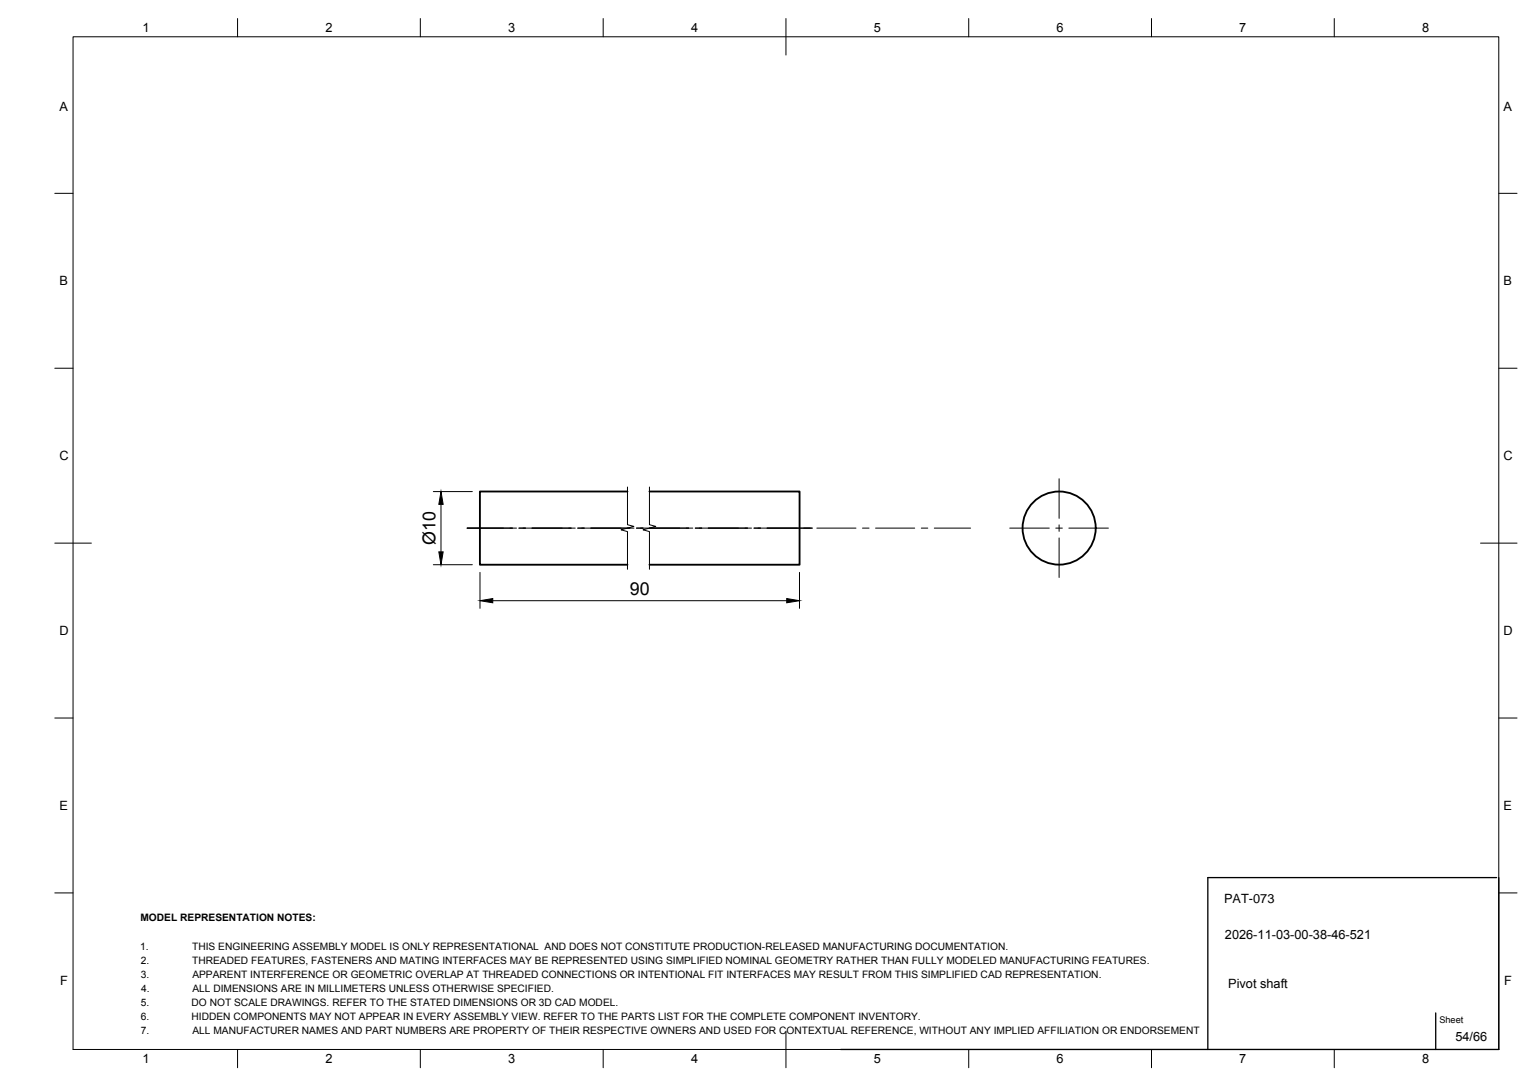
ISO-10303-21;
HEADER;
/* Generated by software containing ST-Developer
 * from STEP Tools, Inc. (www.steptools.com) 
 */

FILE_DESCRIPTION(
/* description */ ('Manual piston pump'),
/* implementation_level */ '2;1');

FILE_NAME(
/* name */ 'Pivot shaft.step',
/* time_stamp */ '2026-11-02T16:54:23-08:00',
/* author */ (''),
/* organization */ (''),
/* preprocessor_version */ 'ST-DEVELOPER v20.2',
/* originating_system */ 'Autodesk Translation Framework v15.17.0.0',
/* authorisation */ '');

FILE_SCHEMA (('AUTOMOTIVE_DESIGN { 1 0 10303 214 3 1 1 }'));
ENDSEC;

DATA;
#10=MECHANICAL_DESIGN_GEOMETRIC_PRESENTATION_REPRESENTATION('',(#744),#19043);
#610=SHAPE_REPRESENTATION_RELATIONSHIP('SRR','None',#19360,#673);
#673=ADVANCED_BREP_SHAPE_REPRESENTATION('',(#812),#19027);
#744=STYLED_ITEM('',(#19664),#812);
#812=MANIFOLD_SOLID_BREP('Body1',#9532);
#1256=CYLINDRICAL_SURFACE('',#11268,0.5);
#1763=FACE_OUTER_BOUND('',#2531,.T.);
#1764=FACE_OUTER_BOUND('',#2532,.T.);
#1765=FACE_OUTER_BOUND('',#2533,.T.);
#2531=EDGE_LOOP('',(#8167,#8168,#8169,#8170));
#2532=EDGE_LOOP('',(#8171));
#2533=EDGE_LOOP('',(#8172));
#3070=CIRCLE('',#11269,0.5);
#3071=CIRCLE('',#11270,0.5);
#3639=LINE('',#18310,#4243);
#4243=VECTOR('',#14041,0.5);
#4990=VERTEX_POINT('',#18307);
#4991=VERTEX_POINT('',#18309);
#6070=EDGE_CURVE('',#4990,#4990,#3070,.T.);
#6071=EDGE_CURVE('',#4990,#4991,#3639,.T.);
#6072=EDGE_CURVE('',#4991,#4991,#3071,.T.);
#8167=ORIENTED_EDGE('',*,*,#6070,.F.);
#8168=ORIENTED_EDGE('',*,*,#6071,.T.);
#8169=ORIENTED_EDGE('',*,*,#6072,.T.);
#8170=ORIENTED_EDGE('',*,*,#6071,.F.);
#8171=ORIENTED_EDGE('',*,*,#6070,.T.);
#8172=ORIENTED_EDGE('',*,*,#6072,.F.);
#8834=PLANE('',#11271);
#8835=PLANE('',#11272);
#9368=ADVANCED_FACE('',(#1763),#1256,.T.);
#9369=ADVANCED_FACE('',(#1764),#8834,.T.);
#9370=ADVANCED_FACE('',(#1765),#8835,.F.);
#9532=CLOSED_SHELL('',(#9368,#9369,#9370));
#11267=AXIS2_PLACEMENT_3D('',#18305,#14035,#14036);
#11268=AXIS2_PLACEMENT_3D('',#18306,#14037,#14038);
#11269=AXIS2_PLACEMENT_3D('',#18308,#14039,#14040);
#11270=AXIS2_PLACEMENT_3D('',#18311,#14042,#14043);
#11271=AXIS2_PLACEMENT_3D('',#18312,#14044,#14045);
#11272=AXIS2_PLACEMENT_3D('',#18313,#14046,#14047);
#14035=DIRECTION('axis',(0.,0.,1.));
#14036=DIRECTION('refdir',(1.,0.,0.));
#14037=DIRECTION('center_axis',(1.,0.,0.));
#14038=DIRECTION('ref_axis',(0.,0.,-1.));
#14039=DIRECTION('center_axis',(1.,0.,0.));
#14040=DIRECTION('ref_axis',(0.,0.,-1.));
#14041=DIRECTION('',(-1.,0.,0.));
#14042=DIRECTION('center_axis',(1.,0.,0.));
#14043=DIRECTION('ref_axis',(0.,0.,-1.));
#14044=DIRECTION('center_axis',(1.,0.,0.));
#14045=DIRECTION('ref_axis',(0.,0.,-1.));
#14046=DIRECTION('center_axis',(1.,0.,0.));
#14047=DIRECTION('ref_axis',(0.,0.,-1.));
#18305=CARTESIAN_POINT('',(0.,0.,0.));
#18306=CARTESIAN_POINT('Origin',(-4.,-4.,10.));
#18307=CARTESIAN_POINT('',(5.,-4.,10.5));
#18308=CARTESIAN_POINT('Origin',(5.,-4.,10.));
#18309=CARTESIAN_POINT('',(-4.,-4.,10.5));
#18310=CARTESIAN_POINT('',(-4.,-4.,10.5));
#18311=CARTESIAN_POINT('Origin',(-4.,-4.,10.));
#18312=CARTESIAN_POINT('Origin',(5.,-4.,10.));
#18313=CARTESIAN_POINT('Origin',(-4.,-4.,10.));
#18956=UNCERTAINTY_MEASURE_WITH_UNIT(LENGTH_MEASURE(0.001),#19044,
'DISTANCE_ACCURACY_VALUE',
'Maximum model space distance between geometric entities at asserted c
onnectivities');
#18972=UNCERTAINTY_MEASURE_WITH_UNIT(LENGTH_MEASURE(0.001),#19044,
'DISTANCE_ACCURACY_VALUE',
'Maximum model space distance between geometric entities at asserted c
onnectivities');
#19027=(
GEOMETRIC_REPRESENTATION_CONTEXT(3)
GLOBAL_UNCERTAINTY_ASSIGNED_CONTEXT((#18956))
GLOBAL_UNIT_ASSIGNED_CONTEXT((#19044,#19046,#19047))
REPRESENTATION_CONTEXT('','3D')
);
#19043=(
GEOMETRIC_REPRESENTATION_CONTEXT(3)
GLOBAL_UNCERTAINTY_ASSIGNED_CONTEXT((#18972))
GLOBAL_UNIT_ASSIGNED_CONTEXT((#19044,#19046,#19047))
REPRESENTATION_CONTEXT('','3D')
);
#19044=(
LENGTH_UNIT()
NAMED_UNIT(*)
SI_UNIT(.CENTI.,.METRE.)
);
#19046=(
NAMED_UNIT(*)
PLANE_ANGLE_UNIT()
SI_UNIT($,.RADIAN.)
);
#19047=(
NAMED_UNIT(*)
SI_UNIT($,.STERADIAN.)
SOLID_ANGLE_UNIT()
);
#19102=SHAPE_DEFINITION_REPRESENTATION(#19259,#19360);
#19259=PRODUCT_DEFINITION_SHAPE('',$,#19431);
#19360=SHAPE_REPRESENTATION('',(#11267),#19027);
#19376=PRODUCT_DEFINITION_CONTEXT('part definition',#19588,'design');
#19431=PRODUCT_DEFINITION('2026-11-03-00-38-46-521','Pivot shaft',#19501,
#19376);
#19501=PRODUCT_DEFINITION_FORMATION('',$,#19644);
#19588=APPLICATION_CONTEXT(
'Core Data for Automotive Mechanical Design Process');
#19589=PRODUCT_CONTEXT('part definition',#19588,'mechanical');
#19644=PRODUCT('2026-11-03-00-38-46-521','Pivot shaft','Pivot shaft',(#19589));
#19664=PRESENTATION_STYLE_ASSIGNMENT((#19670));
#19670=SURFACE_STYLE_USAGE(.BOTH.,#19676);
#19676=SURFACE_SIDE_STYLE('',(#19682));
#19682=SURFACE_STYLE_FILL_AREA(#19688);
#19688=FILL_AREA_STYLE('CAD Library Painted - Steel gray',(#19694));
#19694=FILL_AREA_STYLE_COLOUR('CAD Library Painted - Steel gray',#19700);
#19700=COLOUR_RGB('CAD Library Painted - Steel gray',0.592156862745098,
0.631372549019608,0.67843137254902);
ENDSEC;
END-ISO-10303-21;
